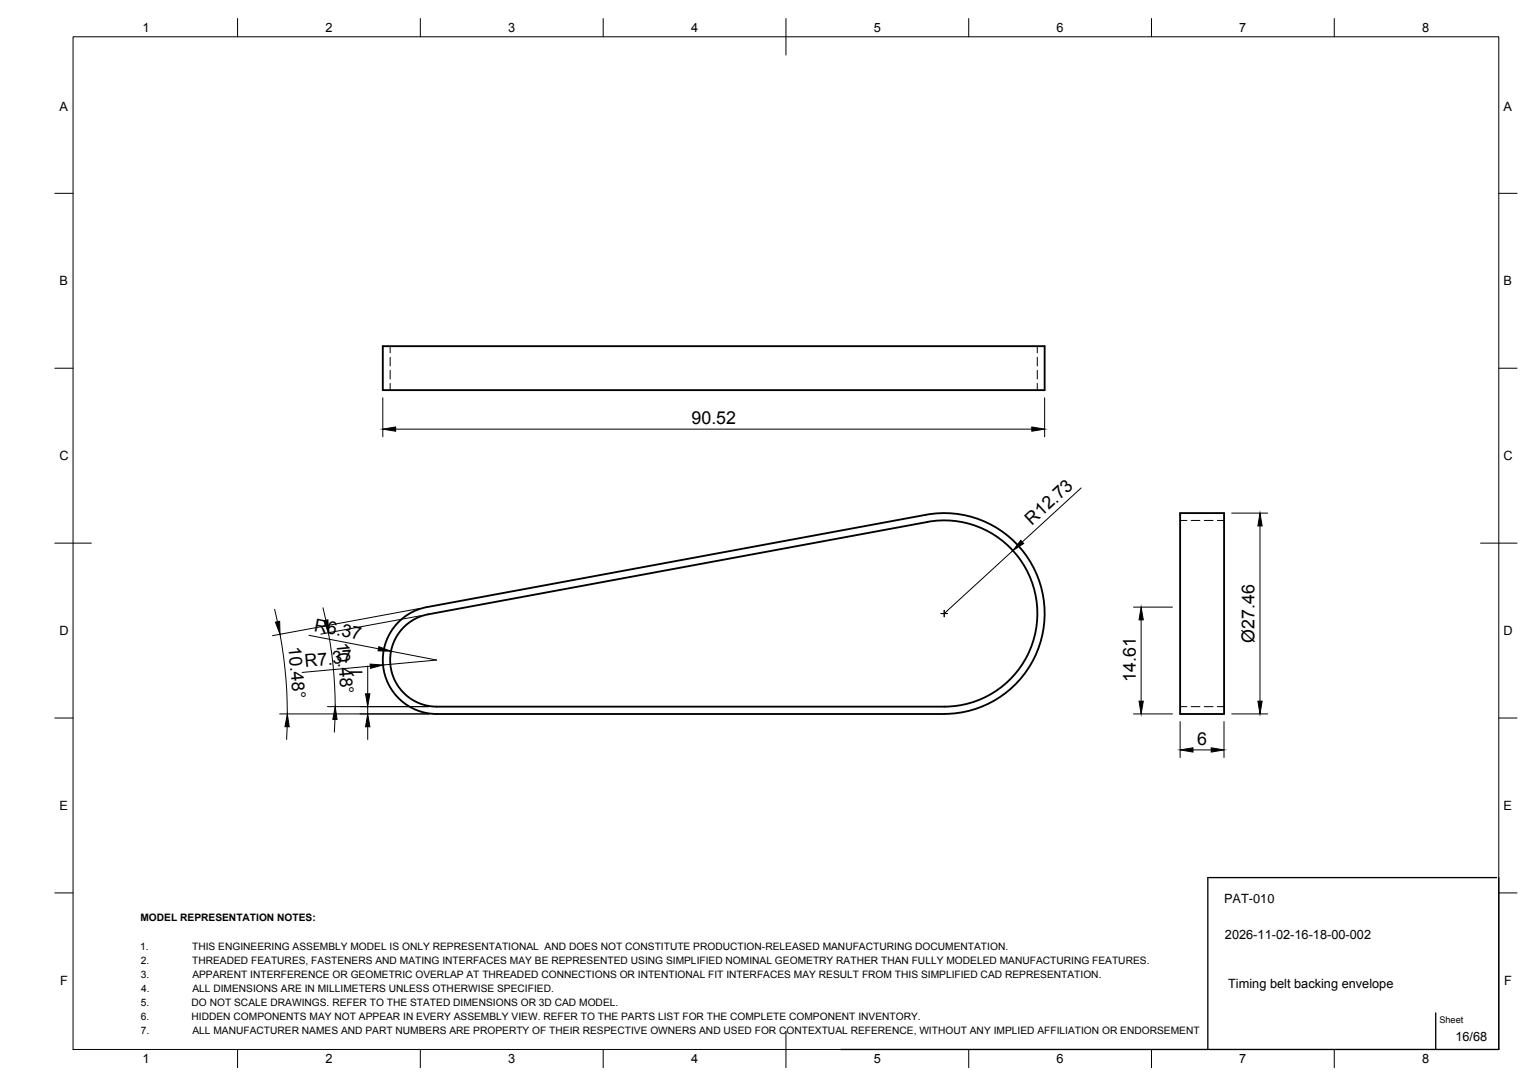
ISO-10303-21;
HEADER;
/* Generated by software containing ST-Developer
 * from STEP Tools, Inc. (www.steptools.com) 
 */

FILE_DESCRIPTION(
/* description */ ('Belt conveyor head drive unit'),
/* implementation_level */ '2;1');

FILE_NAME(
/* name */ 'Timing belt backing envelope.step',
/* time_stamp */ '2026-10-28T03:26:19-07:00',
/* author */ (''),
/* organization */ (''),
/* preprocessor_version */ 'ST-DEVELOPER v20.2',
/* originating_system */ 'Autodesk Translation Framework v15.17.0.0',
/* authorisation */ '');

FILE_SCHEMA (('AUTOMOTIVE_DESIGN { 1 0 10303 214 3 1 1 }'));
ENDSEC;

DATA;
#10=MECHANICAL_DESIGN_GEOMETRIC_PRESENTATION_REPRESENTATION('',(#862),#27069);
#724=SHAPE_REPRESENTATION_RELATIONSHIP('SRR','None',#27368,#793);
#793=ADVANCED_BREP_SHAPE_REPRESENTATION('',(#947),#27010);
#862=STYLED_ITEM('',(#27804),#947);
#947=MANIFOLD_SOLID_BREP('Body1',#13727);
#1091=FACE_BOUND('',#2703,.T.);
#1092=FACE_BOUND('',#2711,.T.);
#1367=PLANE('',#14976);
#1368=PLANE('',#14977);
#1369=PLANE('',#14978);
#1370=PLANE('',#14989);
#1371=PLANE('',#14990);
#1372=PLANE('',#14993);
#1821=FACE_OUTER_BOUND('',#2700,.T.);
#1822=FACE_OUTER_BOUND('',#2701,.T.);
#1823=FACE_OUTER_BOUND('',#2702,.T.);
#1824=FACE_OUTER_BOUND('',#2704,.T.);
#1825=FACE_OUTER_BOUND('',#2705,.T.);
#1826=FACE_OUTER_BOUND('',#2706,.T.);
#1827=FACE_OUTER_BOUND('',#2707,.T.);
#1828=FACE_OUTER_BOUND('',#2708,.T.);
#1829=FACE_OUTER_BOUND('',#2709,.T.);
#1830=FACE_OUTER_BOUND('',#2710,.T.);
#2700=EDGE_LOOP('',(#9816,#9817,#9818,#9819));
#2701=EDGE_LOOP('',(#9820,#9821,#9822,#9823));
#2702=EDGE_LOOP('',(#9824,#9825,#9826,#9827));
#2703=EDGE_LOOP('',(#9828,#9829,#9830,#9831));
#2704=EDGE_LOOP('',(#9832,#9833,#9834,#9835));
#2705=EDGE_LOOP('',(#9836,#9837,#9838,#9839));
#2706=EDGE_LOOP('',(#9840,#9841,#9842,#9843));
#2707=EDGE_LOOP('',(#9844,#9845,#9846,#9847));
#2708=EDGE_LOOP('',(#9848,#9849,#9850,#9851));
#2709=EDGE_LOOP('',(#9852,#9853,#9854,#9855));
#2710=EDGE_LOOP('',(#9856,#9857,#9858,#9859));
#2711=EDGE_LOOP('',(#9860,#9861,#9862,#9863));
#3719=LINE('',#21894,#4511);
#3720=LINE('',#21896,#4512);
#3721=LINE('',#21898,#4513);
#3722=LINE('',#21899,#4514);
#3723=LINE('',#21903,#4515);
#3724=LINE('',#21905,#4516);
#3725=LINE('',#21907,#4517);
#3726=LINE('',#21908,#4518);
#3727=LINE('',#21912,#4519);
#3728=LINE('',#21916,#4520);
#3729=LINE('',#21926,#4521);
#3730=LINE('',#21929,#4522);
#3731=LINE('',#21932,#4523);
#3732=LINE('',#21933,#4524);
#3733=LINE('',#21936,#4525);
#3734=LINE('',#21937,#4526);
#4511=VECTOR('',#17485,1.);
#4512=VECTOR('',#17486,1.);
#4513=VECTOR('',#17487,1.);
#4514=VECTOR('',#17488,1.);
#4515=VECTOR('',#17491,1.);
#4516=VECTOR('',#17492,1.);
#4517=VECTOR('',#17493,1.);
#4518=VECTOR('',#17494,1.);
#4519=VECTOR('',#17497,1.);
#4520=VECTOR('',#17500,1.);
#4521=VECTOR('',#17517,1.);
#4522=VECTOR('',#17520,1.);
#4523=VECTOR('',#17523,1.);
#4524=VECTOR('',#17524,1.);
#4525=VECTOR('',#17527,1.);
#4526=VECTOR('',#17528,1.);
#5290=CIRCLE('',#14979,0.736619772367581);
#5291=CIRCLE('',#14980,1.37323954473516);
#5292=CIRCLE('',#14981,0.636619772367581);
#5293=CIRCLE('',#14982,1.27323954473516);
#5294=CIRCLE('',#14984,0.636619772367581);
#5295=CIRCLE('',#14986,1.27323954473516);
#5296=CIRCLE('',#14988,1.37323954473516);
#5297=CIRCLE('',#14992,0.736619772367581);
#6239=VERTEX_POINT('',#21892);
#6240=VERTEX_POINT('',#21893);
#6241=VERTEX_POINT('',#21895);
#6242=VERTEX_POINT('',#21897);
#6243=VERTEX_POINT('',#21901);
#6244=VERTEX_POINT('',#21902);
#6245=VERTEX_POINT('',#21904);
#6246=VERTEX_POINT('',#21906);
#6247=VERTEX_POINT('',#21910);
#6248=VERTEX_POINT('',#21911);
#6249=VERTEX_POINT('',#21913);
#6250=VERTEX_POINT('',#21915);
#6251=VERTEX_POINT('',#21925);
#6252=VERTEX_POINT('',#21927);
#6253=VERTEX_POINT('',#21931);
#6254=VERTEX_POINT('',#21935);
#7600=EDGE_CURVE('',#6239,#6240,#3719,.T.);
#7601=EDGE_CURVE('',#6241,#6239,#3720,.T.);
#7602=EDGE_CURVE('',#6242,#6241,#3721,.T.);
#7603=EDGE_CURVE('',#6242,#6240,#3722,.T.);
#7604=EDGE_CURVE('',#6243,#6244,#3723,.T.);
#7605=EDGE_CURVE('',#6245,#6243,#3724,.T.);
#7606=EDGE_CURVE('',#6246,#6245,#3725,.T.);
#7607=EDGE_CURVE('',#6244,#6246,#3726,.T.);
#7608=EDGE_CURVE('',#6247,#6248,#3727,.T.);
#7609=EDGE_CURVE('',#6249,#6247,#5290,.T.);
#7610=EDGE_CURVE('',#6250,#6249,#3728,.T.);
#7611=EDGE_CURVE('',#6248,#6250,#5291,.T.);
#7612=EDGE_CURVE('',#6240,#6243,#5292,.T.);
#7613=EDGE_CURVE('',#6244,#6239,#5293,.T.);
#7614=EDGE_CURVE('',#6245,#6242,#5294,.T.);
#7615=EDGE_CURVE('',#6241,#6246,#5295,.T.);
#7616=EDGE_CURVE('',#6250,#6251,#3729,.T.);
#7617=EDGE_CURVE('',#6252,#6251,#5296,.T.);
#7618=EDGE_CURVE('',#6248,#6252,#3730,.T.);
#7619=EDGE_CURVE('',#6249,#6253,#3731,.T.);
#7620=EDGE_CURVE('',#6251,#6253,#3732,.T.);
#7621=EDGE_CURVE('',#6254,#6252,#3733,.T.);
#7622=EDGE_CURVE('',#6247,#6254,#3734,.T.);
#7623=EDGE_CURVE('',#6253,#6254,#5297,.T.);
#9816=ORIENTED_EDGE('',*,*,#7600,.F.);
#9817=ORIENTED_EDGE('',*,*,#7601,.F.);
#9818=ORIENTED_EDGE('',*,*,#7602,.F.);
#9819=ORIENTED_EDGE('',*,*,#7603,.T.);
#9820=ORIENTED_EDGE('',*,*,#7604,.F.);
#9821=ORIENTED_EDGE('',*,*,#7605,.F.);
#9822=ORIENTED_EDGE('',*,*,#7606,.F.);
#9823=ORIENTED_EDGE('',*,*,#7607,.F.);
#9824=ORIENTED_EDGE('',*,*,#7608,.F.);
#9825=ORIENTED_EDGE('',*,*,#7609,.F.);
#9826=ORIENTED_EDGE('',*,*,#7610,.F.);
#9827=ORIENTED_EDGE('',*,*,#7611,.F.);
#9828=ORIENTED_EDGE('',*,*,#7600,.T.);
#9829=ORIENTED_EDGE('',*,*,#7612,.T.);
#9830=ORIENTED_EDGE('',*,*,#7604,.T.);
#9831=ORIENTED_EDGE('',*,*,#7613,.T.);
#9832=ORIENTED_EDGE('',*,*,#7603,.F.);
#9833=ORIENTED_EDGE('',*,*,#7614,.F.);
#9834=ORIENTED_EDGE('',*,*,#7605,.T.);
#9835=ORIENTED_EDGE('',*,*,#7612,.F.);
#9836=ORIENTED_EDGE('',*,*,#7601,.T.);
#9837=ORIENTED_EDGE('',*,*,#7613,.F.);
#9838=ORIENTED_EDGE('',*,*,#7607,.T.);
#9839=ORIENTED_EDGE('',*,*,#7615,.F.);
#9840=ORIENTED_EDGE('',*,*,#7616,.T.);
#9841=ORIENTED_EDGE('',*,*,#7617,.F.);
#9842=ORIENTED_EDGE('',*,*,#7618,.F.);
#9843=ORIENTED_EDGE('',*,*,#7611,.T.);
#9844=ORIENTED_EDGE('',*,*,#7610,.T.);
#9845=ORIENTED_EDGE('',*,*,#7619,.T.);
#9846=ORIENTED_EDGE('',*,*,#7620,.F.);
#9847=ORIENTED_EDGE('',*,*,#7616,.F.);
#9848=ORIENTED_EDGE('',*,*,#7608,.T.);
#9849=ORIENTED_EDGE('',*,*,#7618,.T.);
#9850=ORIENTED_EDGE('',*,*,#7621,.F.);
#9851=ORIENTED_EDGE('',*,*,#7622,.F.);
#9852=ORIENTED_EDGE('',*,*,#7619,.F.);
#9853=ORIENTED_EDGE('',*,*,#7609,.T.);
#9854=ORIENTED_EDGE('',*,*,#7622,.T.);
#9855=ORIENTED_EDGE('',*,*,#7623,.F.);
#9856=ORIENTED_EDGE('',*,*,#7620,.T.);
#9857=ORIENTED_EDGE('',*,*,#7623,.T.);
#9858=ORIENTED_EDGE('',*,*,#7621,.T.);
#9859=ORIENTED_EDGE('',*,*,#7617,.T.);
#9860=ORIENTED_EDGE('',*,*,#7602,.T.);
#9861=ORIENTED_EDGE('',*,*,#7615,.T.);
#9862=ORIENTED_EDGE('',*,*,#7606,.T.);
#9863=ORIENTED_EDGE('',*,*,#7614,.T.);
#12630=CYLINDRICAL_SURFACE('',#14983,0.636619772367581);
#12631=CYLINDRICAL_SURFACE('',#14985,1.27323954473516);
#12632=CYLINDRICAL_SURFACE('',#14987,1.37323954473516);
#12633=CYLINDRICAL_SURFACE('',#14991,0.736619772367581);
#13100=ADVANCED_FACE('',(#1821),#1367,.F.);
#13101=ADVANCED_FACE('',(#1822),#1368,.F.);
#13102=ADVANCED_FACE('',(#1823,#1091),#1369,.F.);
#13103=ADVANCED_FACE('',(#1824),#12630,.F.);
#13104=ADVANCED_FACE('',(#1825),#12631,.F.);
#13105=ADVANCED_FACE('',(#1826),#12632,.T.);
#13106=ADVANCED_FACE('',(#1827),#1370,.T.);
#13107=ADVANCED_FACE('',(#1828),#1371,.T.);
#13108=ADVANCED_FACE('',(#1829),#12633,.T.);
#13109=ADVANCED_FACE('',(#1830,#1092),#1372,.T.);
#13727=CLOSED_SHELL('',(#13100,#13101,#13102,#13103,#13104,#13105,#13106,
#13107,#13108,#13109));
#14975=AXIS2_PLACEMENT_3D('',#21890,#17481,#17482);
#14976=AXIS2_PLACEMENT_3D('',#21891,#17483,#17484);
#14977=AXIS2_PLACEMENT_3D('',#21900,#17489,#17490);
#14978=AXIS2_PLACEMENT_3D('',#21909,#17495,#17496);
#14979=AXIS2_PLACEMENT_3D('',#21914,#17498,#17499);
#14980=AXIS2_PLACEMENT_3D('',#21917,#17501,#17502);
#14981=AXIS2_PLACEMENT_3D('',#21918,#17503,#17504);
#14982=AXIS2_PLACEMENT_3D('',#21919,#17505,#17506);
#14983=AXIS2_PLACEMENT_3D('',#21920,#17507,#17508);
#14984=AXIS2_PLACEMENT_3D('',#21921,#17509,#17510);
#14985=AXIS2_PLACEMENT_3D('',#21922,#17511,#17512);
#14986=AXIS2_PLACEMENT_3D('',#21923,#17513,#17514);
#14987=AXIS2_PLACEMENT_3D('',#21924,#17515,#17516);
#14988=AXIS2_PLACEMENT_3D('',#21928,#17518,#17519);
#14989=AXIS2_PLACEMENT_3D('',#21930,#17521,#17522);
#14990=AXIS2_PLACEMENT_3D('',#21934,#17525,#17526);
#14991=AXIS2_PLACEMENT_3D('',#21938,#17529,#17530);
#14992=AXIS2_PLACEMENT_3D('',#21939,#17531,#17532);
#14993=AXIS2_PLACEMENT_3D('',#21940,#17533,#17534);
#17481=DIRECTION('axis',(0.,0.,1.));
#17482=DIRECTION('refdir',(1.,0.,0.));
#17483=DIRECTION('center_axis',(-0.0913252028230577,0.,-0.99582112215464));
#17484=DIRECTION('ref_axis',(-0.99582112215464,0.,0.0913252028230577));
#17485=DIRECTION('',(-0.99582112215464,0.,0.0913252028230577));
#17486=DIRECTION('',(0.,-1.,0.));
#17487=DIRECTION('',(0.99582112215464,0.,-0.0913252028230577));
#17488=DIRECTION('',(0.,-1.,0.));
#17489=DIRECTION('center_axis',(-0.0913252028230577,0.,0.99582112215464));
#17490=DIRECTION('ref_axis',(0.99582112215464,0.,0.0913252028230577));
#17491=DIRECTION('',(0.99582112215464,0.,0.0913252028230577));
#17492=DIRECTION('',(0.,-1.,0.));
#17493=DIRECTION('',(-0.99582112215464,0.,-0.0913252028230577));
#17494=DIRECTION('',(0.,1.,0.));
#17495=DIRECTION('center_axis',(0.,1.,0.));
#17496=DIRECTION('ref_axis',(1.,0.,0.));
#17497=DIRECTION('',(0.99582112215464,0.,0.091325202823058));
#17498=DIRECTION('center_axis',(0.,1.,0.));
#17499=DIRECTION('ref_axis',(1.,0.,0.));
#17500=DIRECTION('',(-0.99582112215464,0.,0.0913252028230577));
#17501=DIRECTION('center_axis',(0.,1.,0.));
#17502=DIRECTION('ref_axis',(1.,0.,0.));
#17503=DIRECTION('center_axis',(0.,1.,0.));
#17504=DIRECTION('ref_axis',(1.,0.,0.));
#17505=DIRECTION('center_axis',(0.,1.,0.));
#17506=DIRECTION('ref_axis',(1.,0.,0.));
#17507=DIRECTION('center_axis',(0.,1.,0.));
#17508=DIRECTION('ref_axis',(-1.,0.,-1.22464679914735E-16));
#17509=DIRECTION('center_axis',(0.,-1.,0.));
#17510=DIRECTION('ref_axis',(1.,0.,0.));
#17511=DIRECTION('center_axis',(0.,1.,0.));
#17512=DIRECTION('ref_axis',(1.,0.,0.));
#17513=DIRECTION('center_axis',(0.,-1.,0.));
#17514=DIRECTION('ref_axis',(1.,0.,0.));
#17515=DIRECTION('center_axis',(0.,1.,0.));
#17516=DIRECTION('ref_axis',(1.,0.,0.));
#17517=DIRECTION('',(0.,1.,0.));
#17518=DIRECTION('center_axis',(0.,1.,0.));
#17519=DIRECTION('ref_axis',(1.,0.,0.));
#17520=DIRECTION('',(0.,1.,0.));
#17521=DIRECTION('center_axis',(-0.0913252028230577,0.,-0.99582112215464));
#17522=DIRECTION('ref_axis',(-0.99582112215464,0.,0.0913252028230577));
#17523=DIRECTION('',(0.,1.,0.));
#17524=DIRECTION('',(-0.99582112215464,0.,0.0913252028230577));
#17525=DIRECTION('center_axis',(-0.091325202823058,0.,0.99582112215464));
#17526=DIRECTION('ref_axis',(0.99582112215464,0.,0.091325202823058));
#17527=DIRECTION('',(0.99582112215464,0.,0.091325202823058));
#17528=DIRECTION('',(0.,1.,0.));
#17529=DIRECTION('center_axis',(0.,1.,0.));
#17530=DIRECTION('ref_axis',(-1.,0.,-1.22464679914735E-16));
#17531=DIRECTION('center_axis',(0.,1.,0.));
#17532=DIRECTION('ref_axis',(1.,0.,0.));
#17533=DIRECTION('center_axis',(0.,1.,0.));
#17534=DIRECTION('ref_axis',(1.,0.,0.));
#21890=CARTESIAN_POINT('',(0.,0.,0.));
#21891=CARTESIAN_POINT('Origin',(6.85463117051588,-3.5,5.73208116779017));
#21892=CARTESIAN_POINT('',(6.85463117051588,-3.425,5.73208116779017));
#21893=CARTESIAN_POINT('',(-0.0581394298326381,-3.425,6.36604058389508));
#21894=CARTESIAN_POINT('',(3.39824587034162,-3.425,6.04906087584262));
#21895=CARTESIAN_POINT('',(6.85463117051588,-2.825,5.73208116779017));
#21896=CARTESIAN_POINT('',(6.85463117051588,-3.5,5.73208116779017));
#21897=CARTESIAN_POINT('',(-0.0581394298326381,-2.825,6.36604058389508));
#21898=CARTESIAN_POINT('',(3.39824587034162,-2.825,6.04906087584262));
#21899=CARTESIAN_POINT('',(-0.0581394298326381,-3.5,6.36604058389508));
#21900=CARTESIAN_POINT('Origin',(-0.0581394298326382,-3.5,7.63395941610492));
#21901=CARTESIAN_POINT('',(-0.0581394298326382,-3.425,7.63395941610492));
#21902=CARTESIAN_POINT('',(6.85463117051588,-3.425,8.26791883220983));
#21903=CARTESIAN_POINT('',(-0.0581394298326382,-3.425,7.63395941610492));
#21904=CARTESIAN_POINT('',(-0.0581394298326382,-2.825,7.63395941610492));
#21905=CARTESIAN_POINT('',(-0.0581394298326382,-3.5,7.63395941610492));
#21906=CARTESIAN_POINT('',(6.85463117051588,-2.825,8.26791883220983));
#21907=CARTESIAN_POINT('',(-0.0581394298326382,-2.825,7.63395941610492));
#21908=CARTESIAN_POINT('',(6.85463117051588,-3.5,8.26791883220983));
#21909=CARTESIAN_POINT('Origin',(0.,-3.425,7.));
#21910=CARTESIAN_POINT('',(-0.067271950114944,-3.425,7.73354152832038));
#21911=CARTESIAN_POINT('',(6.84549865023357,-3.425,8.3675009444253));
#21912=CARTESIAN_POINT('',(-0.067271950114944,-3.425,7.73354152832038));
#21913=CARTESIAN_POINT('',(-0.067271950114944,-3.425,6.26645847167962));
#21914=CARTESIAN_POINT('Origin',(0.,-3.425,7.));
#21915=CARTESIAN_POINT('',(6.84549865023357,-3.425,5.6324990555747));
#21916=CARTESIAN_POINT('',(6.84549865023357,-3.425,5.6324990555747));
#21917=CARTESIAN_POINT('Origin',(6.97091003018116,-3.425,7.));
#21918=CARTESIAN_POINT('Origin',(0.,-3.425,7.));
#21919=CARTESIAN_POINT('Origin',(6.97091003018116,-3.425,7.));
#21920=CARTESIAN_POINT('Origin',(0.,-3.5,7.));
#21921=CARTESIAN_POINT('Origin',(0.,-2.825,7.));
#21922=CARTESIAN_POINT('Origin',(6.97091003018116,-3.5,7.));
#21923=CARTESIAN_POINT('Origin',(6.97091003018116,-2.825,7.));
#21924=CARTESIAN_POINT('Origin',(6.97091003018116,-3.425,7.));
#21925=CARTESIAN_POINT('',(6.84549865023357,-2.825,5.6324990555747));
#21926=CARTESIAN_POINT('',(6.84549865023357,-3.425,5.6324990555747));
#21927=CARTESIAN_POINT('',(6.84549865023357,-2.825,8.3675009444253));
#21928=CARTESIAN_POINT('Origin',(6.97091003018116,-2.825,7.));
#21929=CARTESIAN_POINT('',(6.84549865023357,-3.425,8.3675009444253));
#21930=CARTESIAN_POINT('Origin',(6.84549865023357,-3.425,5.6324990555747));
#21931=CARTESIAN_POINT('',(-0.067271950114944,-2.825,6.26645847167962));
#21932=CARTESIAN_POINT('',(-0.0672719501149439,-3.425,6.26645847167962));
#21933=CARTESIAN_POINT('',(6.84549865023357,-2.825,5.6324990555747));
#21934=CARTESIAN_POINT('Origin',(-0.067271950114944,-3.425,7.73354152832038));
#21935=CARTESIAN_POINT('',(-0.067271950114944,-2.825,7.73354152832038));
#21936=CARTESIAN_POINT('',(-0.067271950114944,-2.825,7.73354152832038));
#21937=CARTESIAN_POINT('',(-0.0672719501149441,-3.425,7.73354152832038));
#21938=CARTESIAN_POINT('Origin',(0.,-3.425,7.));
#21939=CARTESIAN_POINT('Origin',(0.,-2.825,7.));
#21940=CARTESIAN_POINT('Origin',(0.,-2.825,7.));
#26933=UNCERTAINTY_MEASURE_WITH_UNIT(LENGTH_MEASURE(0.001),#27070,
'DISTANCE_ACCURACY_VALUE',
'Maximum model space distance between geometric entities at asserted c
onnectivities');
#26992=UNCERTAINTY_MEASURE_WITH_UNIT(LENGTH_MEASURE(0.001),#27070,
'DISTANCE_ACCURACY_VALUE',
'Maximum model space distance between geometric entities at asserted c
onnectivities');
#27010=(
GEOMETRIC_REPRESENTATION_CONTEXT(3)
GLOBAL_UNCERTAINTY_ASSIGNED_CONTEXT((#26933))
GLOBAL_UNIT_ASSIGNED_CONTEXT((#27070,#27072,#27073))
REPRESENTATION_CONTEXT('','3D')
);
#27069=(
GEOMETRIC_REPRESENTATION_CONTEXT(3)
GLOBAL_UNCERTAINTY_ASSIGNED_CONTEXT((#26992))
GLOBAL_UNIT_ASSIGNED_CONTEXT((#27070,#27072,#27073))
REPRESENTATION_CONTEXT('','3D')
);
#27070=(
LENGTH_UNIT()
NAMED_UNIT(*)
SI_UNIT(.CENTI.,.METRE.)
);
#27072=(
NAMED_UNIT(*)
PLANE_ANGLE_UNIT()
SI_UNIT($,.RADIAN.)
);
#27073=(
NAMED_UNIT(*)
SI_UNIT($,.STERADIAN.)
SOLID_ANGLE_UNIT()
);
#27091=SHAPE_DEFINITION_REPRESENTATION(#27167,#27368);
#27167=PRODUCT_DEFINITION_SHAPE('',$,#27445);
#27368=SHAPE_REPRESENTATION('',(#14975),#27010);
#27427=PRODUCT_DEFINITION_CONTEXT('part definition',#27657,'design');
#27445=PRODUCT_DEFINITION('Timing belt backing envelope',
'Timing belt backing envelope',#27521,#27427);
#27521=PRODUCT_DEFINITION_FORMATION('',$,#27676);
#27657=APPLICATION_CONTEXT(
'Core Data for Automotive Mechanical Design Process');
#27658=PRODUCT_CONTEXT('part definition',#27657,'mechanical');
#27676=PRODUCT('Timing belt backing envelope',
'Timing belt backing envelope','Timing belt backing envelope',(#27658));
#27798=COLOUR_RGB('Black',0.12,0.14,0.17);
#27799=FILL_AREA_STYLE_COLOUR('',#27798);
#27800=FILL_AREA_STYLE('',(#27799));
#27801=SURFACE_STYLE_FILL_AREA(#27800);
#27802=SURFACE_SIDE_STYLE('',(#27801));
#27803=SURFACE_STYLE_USAGE(.BOTH.,#27802);
#27804=PRESENTATION_STYLE_ASSIGNMENT((#27803));
ENDSEC;
END-ISO-10303-21;
